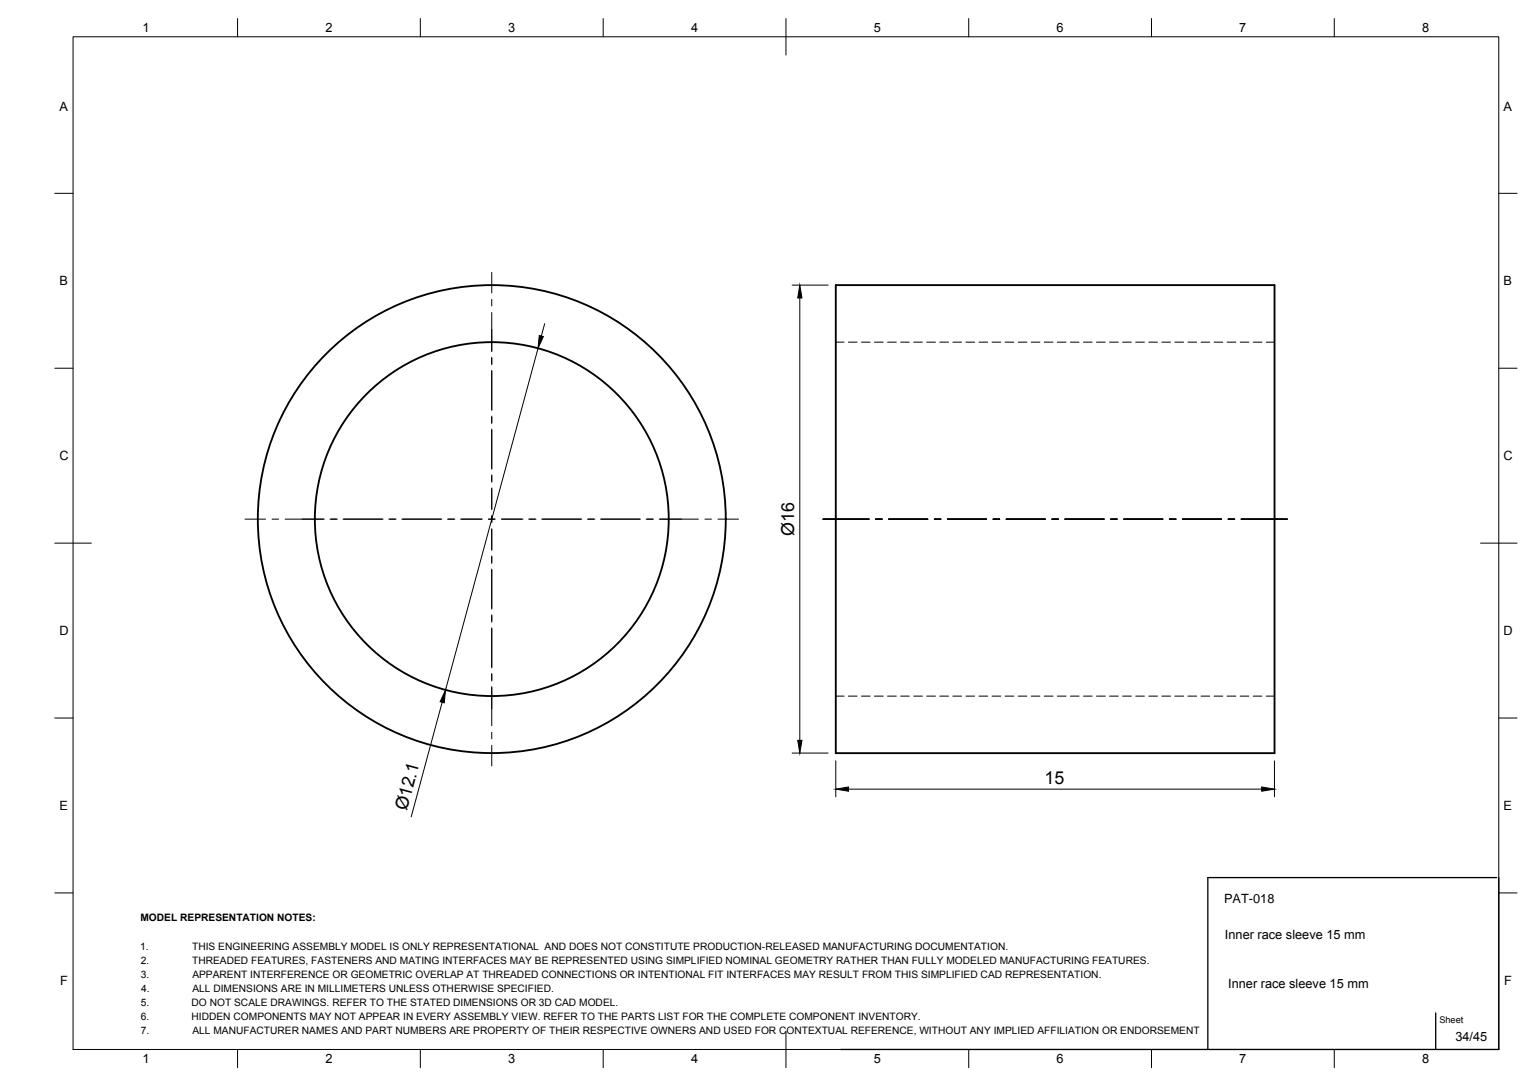
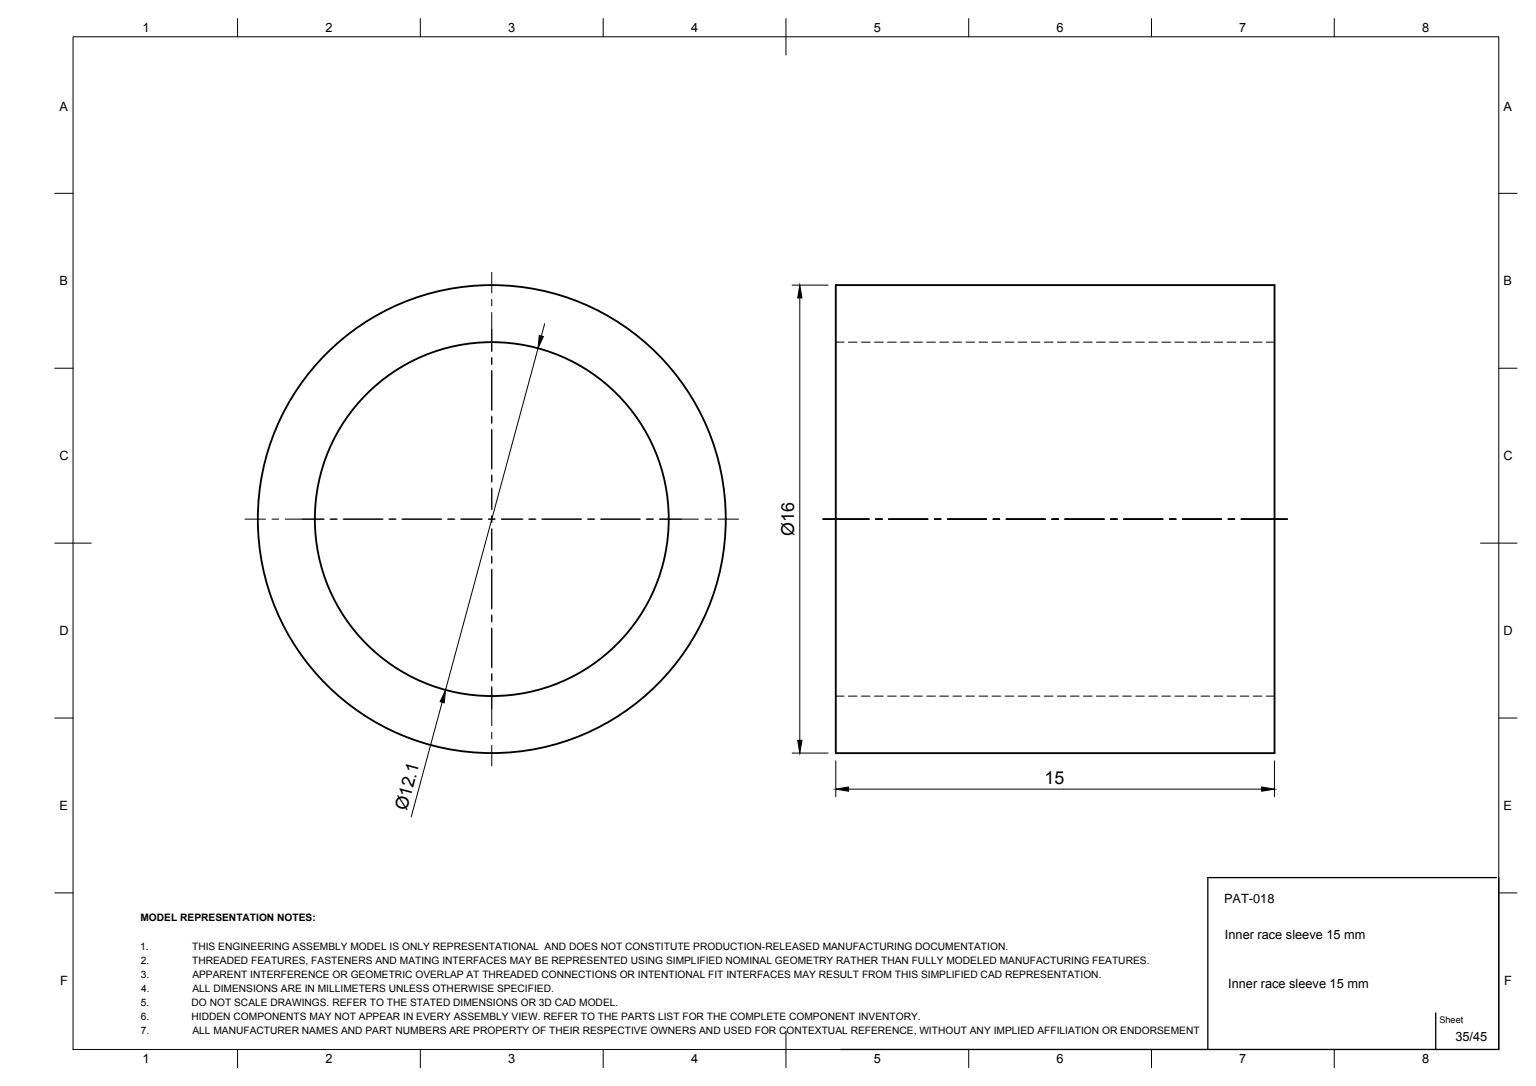
ISO-10303-21;
HEADER;
/* Generated by software containing ST-Developer
 * from STEP Tools, Inc. (www.steptools.com) 
 */

FILE_DESCRIPTION(
/* description */ ('Cam-driven reciprocating slide'),
/* implementation_level */ '2;1');

FILE_NAME(
/* name */ 'Inner race sleeve 15 mm.step',
/* time_stamp */ '2026-10-28T03:25:20-07:00',
/* author */ (''),
/* organization */ (''),
/* preprocessor_version */ 'ST-DEVELOPER v20.2',
/* originating_system */ 'Autodesk Translation Framework v15.17.0.0',
/* authorisation */ '');

FILE_SCHEMA (('AUTOMOTIVE_DESIGN { 1 0 10303 214 3 1 1 }'));
ENDSEC;

DATA;
#10=MECHANICAL_DESIGN_GEOMETRIC_PRESENTATION_REPRESENTATION('',(#454),#13277);
#373=SHAPE_REPRESENTATION_RELATIONSHIP('SRR','None',#13469,#410);
#410=ADVANCED_BREP_SHAPE_REPRESENTATION('',(#496),#13264);
#454=STYLED_ITEM('',(#13720),#496);
#496=MANIFOLD_SOLID_BREP('Body1',#6432);
#648=FACE_BOUND('',#1706,.T.);
#649=FACE_BOUND('',#1708,.T.);
#837=PLANE('',#7438);
#838=PLANE('',#7439);
#1183=FACE_OUTER_BOUND('',#1703,.T.);
#1184=FACE_OUTER_BOUND('',#1704,.T.);
#1185=FACE_OUTER_BOUND('',#1705,.T.);
#1186=FACE_OUTER_BOUND('',#1707,.T.);
#1703=EDGE_LOOP('',(#5516,#5517,#5518,#5519));
#1704=EDGE_LOOP('',(#5520,#5521,#5522,#5523));
#1705=EDGE_LOOP('',(#5524));
#1706=EDGE_LOOP('',(#5525));
#1707=EDGE_LOOP('',(#5526));
#1708=EDGE_LOOP('',(#5527));
#2148=LINE('',#12709,#2587);
#2149=LINE('',#12715,#2588);
#2587=VECTOR('',#9146,0.605);
#2588=VECTOR('',#9153,0.8);
#2971=CIRCLE('',#7433,0.605);
#2972=CIRCLE('',#7434,0.605);
#2973=CIRCLE('',#7436,0.8);
#2974=CIRCLE('',#7437,0.8);
#3434=VERTEX_POINT('',#12706);
#3435=VERTEX_POINT('',#12708);
#3436=VERTEX_POINT('',#12712);
#3437=VERTEX_POINT('',#12714);
#4148=EDGE_CURVE('',#3434,#3434,#2971,.T.);
#4149=EDGE_CURVE('',#3434,#3435,#2148,.T.);
#4150=EDGE_CURVE('',#3435,#3435,#2972,.T.);
#4151=EDGE_CURVE('',#3436,#3436,#2973,.T.);
#4152=EDGE_CURVE('',#3436,#3437,#2149,.T.);
#4153=EDGE_CURVE('',#3437,#3437,#2974,.T.);
#5516=ORIENTED_EDGE('',*,*,#4148,.F.);
#5517=ORIENTED_EDGE('',*,*,#4149,.T.);
#5518=ORIENTED_EDGE('',*,*,#4150,.T.);
#5519=ORIENTED_EDGE('',*,*,#4149,.F.);
#5520=ORIENTED_EDGE('',*,*,#4151,.F.);
#5521=ORIENTED_EDGE('',*,*,#4152,.T.);
#5522=ORIENTED_EDGE('',*,*,#4153,.T.);
#5523=ORIENTED_EDGE('',*,*,#4152,.F.);
#5524=ORIENTED_EDGE('',*,*,#4151,.T.);
#5525=ORIENTED_EDGE('',*,*,#4148,.T.);
#5526=ORIENTED_EDGE('',*,*,#4153,.F.);
#5527=ORIENTED_EDGE('',*,*,#4150,.F.);
#5990=CYLINDRICAL_SURFACE('',#7432,0.605);
#5991=CYLINDRICAL_SURFACE('',#7435,0.8);
#6301=ADVANCED_FACE('',(#1183),#5990,.F.);
#6302=ADVANCED_FACE('',(#1184),#5991,.T.);
#6303=ADVANCED_FACE('',(#1185,#648),#837,.T.);
#6304=ADVANCED_FACE('',(#1186,#649),#838,.F.);
#6432=CLOSED_SHELL('',(#6301,#6302,#6303,#6304));
#7431=AXIS2_PLACEMENT_3D('',#12704,#9140,#9141);
#7432=AXIS2_PLACEMENT_3D('',#12705,#9142,#9143);
#7433=AXIS2_PLACEMENT_3D('',#12707,#9144,#9145);
#7434=AXIS2_PLACEMENT_3D('',#12710,#9147,#9148);
#7435=AXIS2_PLACEMENT_3D('',#12711,#9149,#9150);
#7436=AXIS2_PLACEMENT_3D('',#12713,#9151,#9152);
#7437=AXIS2_PLACEMENT_3D('',#12716,#9154,#9155);
#7438=AXIS2_PLACEMENT_3D('',#12717,#9156,#9157);
#7439=AXIS2_PLACEMENT_3D('',#12718,#9158,#9159);
#9140=DIRECTION('axis',(0.,0.,1.));
#9141=DIRECTION('refdir',(1.,0.,0.));
#9142=DIRECTION('center_axis',(0.,1.,0.));
#9143=DIRECTION('ref_axis',(1.,0.,0.));
#9144=DIRECTION('center_axis',(0.,-1.,0.));
#9145=DIRECTION('ref_axis',(1.,0.,0.));
#9146=DIRECTION('',(0.,-1.,0.));
#9147=DIRECTION('center_axis',(0.,-1.,0.));
#9148=DIRECTION('ref_axis',(1.,0.,0.));
#9149=DIRECTION('center_axis',(0.,1.,0.));
#9150=DIRECTION('ref_axis',(1.,0.,0.));
#9151=DIRECTION('center_axis',(0.,1.,0.));
#9152=DIRECTION('ref_axis',(1.,0.,0.));
#9153=DIRECTION('',(0.,-1.,0.));
#9154=DIRECTION('center_axis',(0.,1.,0.));
#9155=DIRECTION('ref_axis',(1.,0.,0.));
#9156=DIRECTION('center_axis',(0.,1.,0.));
#9157=DIRECTION('ref_axis',(1.,0.,0.));
#9158=DIRECTION('center_axis',(0.,1.,0.));
#9159=DIRECTION('ref_axis',(1.,0.,0.));
#12704=CARTESIAN_POINT('',(0.,0.,0.));
#12705=CARTESIAN_POINT('Origin',(0.,-4.5,4.));
#12706=CARTESIAN_POINT('',(-0.605,-3.,4.));
#12707=CARTESIAN_POINT('Origin',(0.,-3.,4.));
#12708=CARTESIAN_POINT('',(-0.605,-4.5,4.));
#12709=CARTESIAN_POINT('',(-0.605,-4.5,4.));
#12710=CARTESIAN_POINT('Origin',(0.,-4.5,4.));
#12711=CARTESIAN_POINT('Origin',(0.,-4.5,4.));
#12712=CARTESIAN_POINT('',(-0.8,-3.,4.));
#12713=CARTESIAN_POINT('Origin',(0.,-3.,4.));
#12714=CARTESIAN_POINT('',(-0.8,-4.5,4.));
#12715=CARTESIAN_POINT('',(-0.8,-4.5,4.));
#12716=CARTESIAN_POINT('Origin',(0.,-4.5,4.));
#12717=CARTESIAN_POINT('Origin',(0.,-3.,4.));
#12718=CARTESIAN_POINT('Origin',(0.,-4.5,4.));
#13220=UNCERTAINTY_MEASURE_WITH_UNIT(LENGTH_MEASURE(0.001),#13278,
'DISTANCE_ACCURACY_VALUE',
'Maximum model space distance between geometric entities at asserted c
onnectivities');
#13233=UNCERTAINTY_MEASURE_WITH_UNIT(LENGTH_MEASURE(0.001),#13278,
'DISTANCE_ACCURACY_VALUE',
'Maximum model space distance between geometric entities at asserted c
onnectivities');
#13264=(
GEOMETRIC_REPRESENTATION_CONTEXT(3)
GLOBAL_UNCERTAINTY_ASSIGNED_CONTEXT((#13220))
GLOBAL_UNIT_ASSIGNED_CONTEXT((#13278,#13280,#13281))
REPRESENTATION_CONTEXT('','3D')
);
#13277=(
GEOMETRIC_REPRESENTATION_CONTEXT(3)
GLOBAL_UNCERTAINTY_ASSIGNED_CONTEXT((#13233))
GLOBAL_UNIT_ASSIGNED_CONTEXT((#13278,#13280,#13281))
REPRESENTATION_CONTEXT('','3D')
);
#13278=(
LENGTH_UNIT()
NAMED_UNIT(*)
SI_UNIT(.CENTI.,.METRE.)
);
#13280=(
NAMED_UNIT(*)
PLANE_ANGLE_UNIT()
SI_UNIT($,.RADIAN.)
);
#13281=(
NAMED_UNIT(*)
SI_UNIT($,.STERADIAN.)
SOLID_ANGLE_UNIT()
);
#13312=SHAPE_DEFINITION_REPRESENTATION(#13362,#13469);
#13362=PRODUCT_DEFINITION_SHAPE('',$,#13513);
#13469=SHAPE_REPRESENTATION('',(#7431),#13264);
#13482=PRODUCT_DEFINITION_CONTEXT('part definition',#13613,'design');
#13513=PRODUCT_DEFINITION('Inner race sleeve 15 mm',
'Inner race sleeve 15 mm',#13556,#13482);
#13556=PRODUCT_DEFINITION_FORMATION('',$,#13645);
#13613=APPLICATION_CONTEXT(
'Core Data for Automotive Mechanical Design Process');
#13614=PRODUCT_CONTEXT('part definition',#13613,'mechanical');
#13645=PRODUCT('Inner race sleeve 15 mm','Inner race sleeve 15 mm',
'Inner race sleeve 15 mm',(#13614));
#13714=COLOUR_RGB('Grey',0.48,0.52,0.57);
#13715=FILL_AREA_STYLE_COLOUR('',#13714);
#13716=FILL_AREA_STYLE('',(#13715));
#13717=SURFACE_STYLE_FILL_AREA(#13716);
#13718=SURFACE_SIDE_STYLE('',(#13717));
#13719=SURFACE_STYLE_USAGE(.BOTH.,#13718);
#13720=PRESENTATION_STYLE_ASSIGNMENT((#13719));
ENDSEC;
END-ISO-10303-21;
